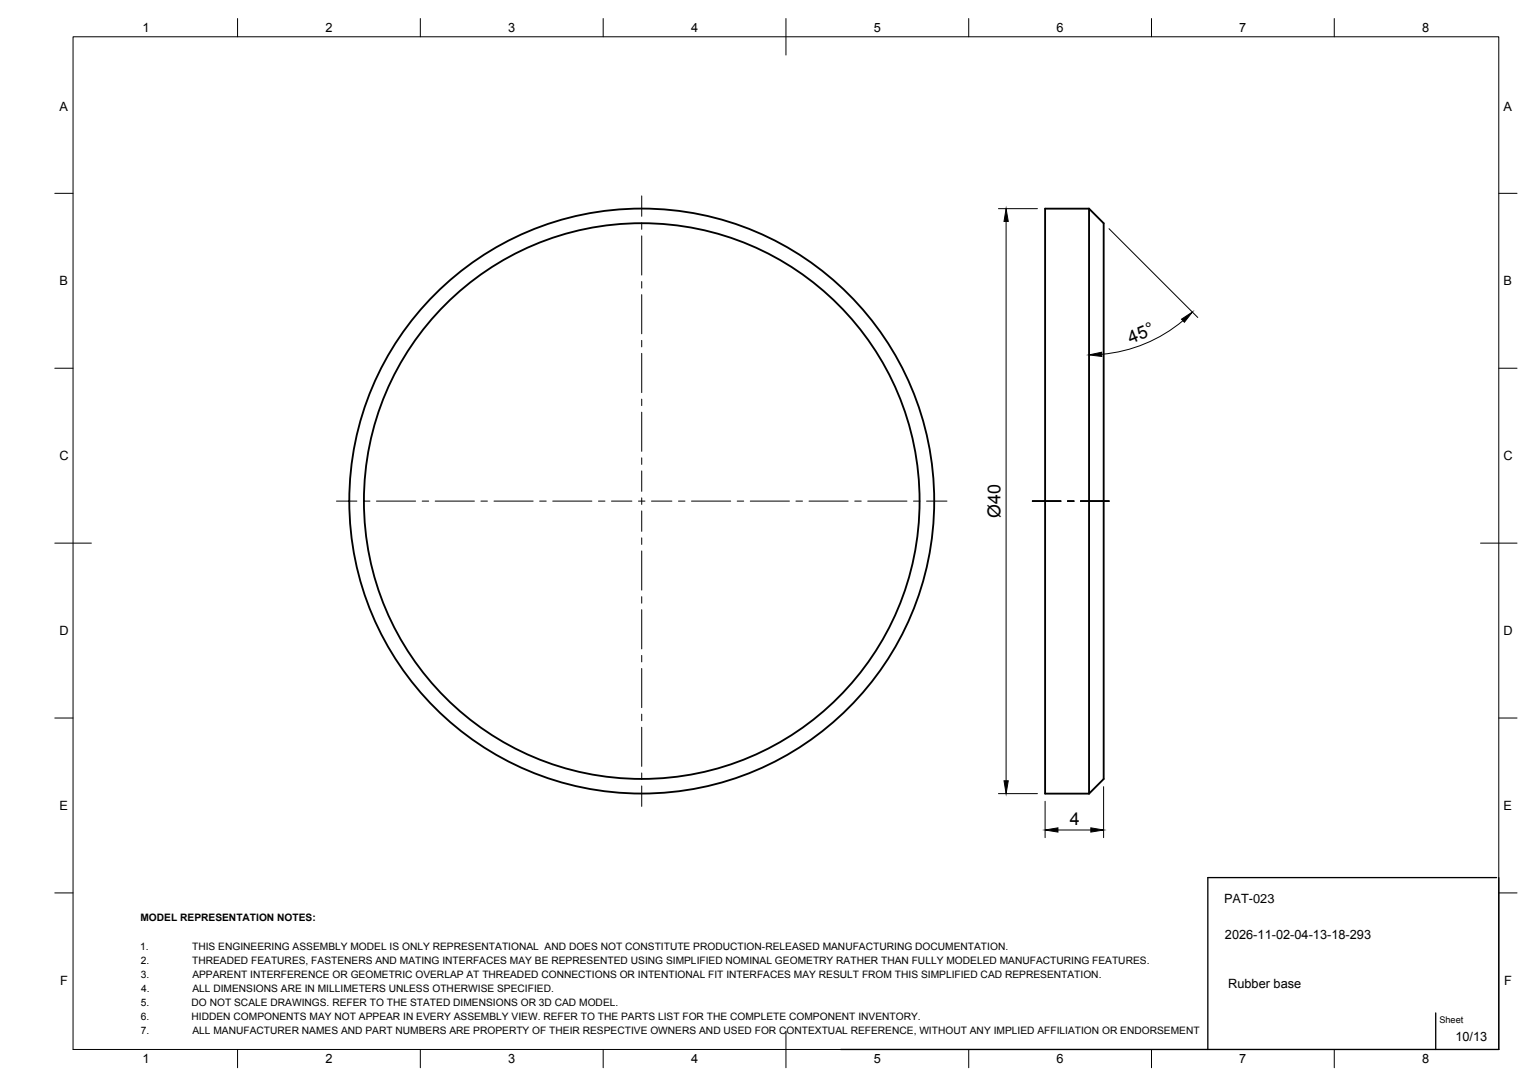
ISO-10303-21;
HEADER;
/* Generated by software containing ST-Developer
 * from STEP Tools, Inc. (www.steptools.com) 
 */

FILE_DESCRIPTION(
/* description */ ('PAT-023'),
/* implementation_level */ '2;1');

FILE_NAME(
/* name */ 'Rubber base.step',
/* time_stamp */ '2026-10-29T15:47:46-07:00',
/* author */ (''),
/* organization */ (''),
/* preprocessor_version */ 'ST-DEVELOPER v20.2',
/* originating_system */ 'Autodesk Translation Framework v15.17.0.0',
/* authorisation */ '');

FILE_SCHEMA (('AUTOMOTIVE_DESIGN { 1 0 10303 214 3 1 1 }'));
ENDSEC;

DATA;
#10=MECHANICAL_DESIGN_GEOMETRIC_PRESENTATION_REPRESENTATION('',(#87),#3773);
#63=CONICAL_SURFACE('',#2387,1.95,0.785398163397449);
#71=SHAPE_REPRESENTATION_RELATIONSHIP('SRR','None',#3819,#79);
#79=ADVANCED_BREP_SHAPE_REPRESENTATION('',(#95),#3767);
#87=STYLED_ITEM('',(#3953),#95);
#95=MANIFOLD_SOLID_BREP('Body1',#2240);
#150=PLANE('',#2385);
#151=PLANE('',#2391);
#256=FACE_OUTER_BOUND('',#384,.T.);
#257=FACE_OUTER_BOUND('',#385,.T.);
#258=FACE_OUTER_BOUND('',#386,.T.);
#259=FACE_OUTER_BOUND('',#387,.T.);
#384=EDGE_LOOP('',(#1711));
#385=EDGE_LOOP('',(#1712,#1713,#1714,#1715));
#386=EDGE_LOOP('',(#1716,#1717,#1718,#1719));
#387=EDGE_LOOP('',(#1720));
#562=LINE('',#3314,#826);
#563=LINE('',#3318,#827);
#826=VECTOR('',#2703,1.95);
#827=VECTOR('',#2708,2.);
#1005=CIRCLE('',#2386,1.9);
#1006=CIRCLE('',#2388,2.);
#1007=CIRCLE('',#2390,2.);
#1089=VERTEX_POINT('',#3309);
#1090=VERTEX_POINT('',#3312);
#1091=VERTEX_POINT('',#3316);
#1318=EDGE_CURVE('',#1089,#1089,#1005,.T.);
#1319=EDGE_CURVE('',#1090,#1090,#1006,.T.);
#1320=EDGE_CURVE('',#1090,#1089,#562,.T.);
#1321=EDGE_CURVE('',#1091,#1091,#1007,.T.);
#1322=EDGE_CURVE('',#1091,#1090,#563,.T.);
#1711=ORIENTED_EDGE('',*,*,#1318,.F.);
#1712=ORIENTED_EDGE('',*,*,#1319,.F.);
#1713=ORIENTED_EDGE('',*,*,#1320,.T.);
#1714=ORIENTED_EDGE('',*,*,#1318,.T.);
#1715=ORIENTED_EDGE('',*,*,#1320,.F.);
#1716=ORIENTED_EDGE('',*,*,#1321,.F.);
#1717=ORIENTED_EDGE('',*,*,#1322,.T.);
#1718=ORIENTED_EDGE('',*,*,#1319,.T.);
#1719=ORIENTED_EDGE('',*,*,#1322,.F.);
#1720=ORIENTED_EDGE('',*,*,#1321,.T.);
#2112=CYLINDRICAL_SURFACE('',#2389,2.);
#2156=ADVANCED_FACE('',(#256),#150,.T.);
#2157=ADVANCED_FACE('',(#257),#63,.T.);
#2158=ADVANCED_FACE('',(#258),#2112,.T.);
#2159=ADVANCED_FACE('',(#259),#151,.T.);
#2240=CLOSED_SHELL('',(#2156,#2157,#2158,#2159));
#2384=AXIS2_PLACEMENT_3D('',#3307,#2693,#2694);
#2385=AXIS2_PLACEMENT_3D('',#3308,#2695,#2696);
#2386=AXIS2_PLACEMENT_3D('',#3310,#2697,#2698);
#2387=AXIS2_PLACEMENT_3D('',#3311,#2699,#2700);
#2388=AXIS2_PLACEMENT_3D('',#3313,#2701,#2702);
#2389=AXIS2_PLACEMENT_3D('',#3315,#2704,#2705);
#2390=AXIS2_PLACEMENT_3D('',#3317,#2706,#2707);
#2391=AXIS2_PLACEMENT_3D('',#3319,#2709,#2710);
#2693=DIRECTION('axis',(0.,0.,1.));
#2694=DIRECTION('refdir',(1.,0.,0.));
#2695=DIRECTION('center_axis',(0.,0.,-1.));
#2696=DIRECTION('ref_axis',(-1.,0.,0.));
#2697=DIRECTION('center_axis',(0.,0.,1.));
#2698=DIRECTION('ref_axis',(1.,0.,0.));
#2699=DIRECTION('center_axis',(0.,0.,1.));
#2700=DIRECTION('ref_axis',(1.,0.,0.));
#2701=DIRECTION('center_axis',(0.,0.,1.));
#2702=DIRECTION('ref_axis',(1.,0.,0.));
#2703=DIRECTION('',(0.707106781186548,8.65956056235494E-17,-0.707106781186547));
#2704=DIRECTION('center_axis',(0.,0.,1.));
#2705=DIRECTION('ref_axis',(1.,0.,0.));
#2706=DIRECTION('center_axis',(0.,0.,1.));
#2707=DIRECTION('ref_axis',(1.,0.,0.));
#2708=DIRECTION('',(0.,0.,-1.));
#2709=DIRECTION('center_axis',(0.,0.,1.));
#2710=DIRECTION('ref_axis',(1.,0.,0.));
#3307=CARTESIAN_POINT('',(0.,0.,0.));
#3308=CARTESIAN_POINT('Origin',(1.9,0.,0.));
#3309=CARTESIAN_POINT('',(-1.9,-2.32682891837997E-16,-4.16333634234434E-17));
#3310=CARTESIAN_POINT('Origin',(0.,0.,0.));
#3311=CARTESIAN_POINT('Origin',(0.,0.,0.05));
#3312=CARTESIAN_POINT('',(-2.,-2.44929359829471E-16,0.1));
#3313=CARTESIAN_POINT('Origin',(0.,0.,0.1));
#3314=CARTESIAN_POINT('',(-1.95,-2.38806125833734E-16,0.05));
#3315=CARTESIAN_POINT('Origin',(0.,0.,0.25));
#3316=CARTESIAN_POINT('',(-2.,-2.44929359829471E-16,0.4));
#3317=CARTESIAN_POINT('Origin',(0.,0.,0.4));
#3318=CARTESIAN_POINT('',(-2.,-2.44929359829471E-16,0.25));
#3319=CARTESIAN_POINT('Origin',(0.,0.,0.4));
#3754=UNCERTAINTY_MEASURE_WITH_UNIT(LENGTH_MEASURE(0.001),#3774,
'DISTANCE_ACCURACY_VALUE',
'Maximum model space distance between geometric entities at asserted c
onnectivities');
#3760=UNCERTAINTY_MEASURE_WITH_UNIT(LENGTH_MEASURE(0.001),#3774,
'DISTANCE_ACCURACY_VALUE',
'Maximum model space distance between geometric entities at asserted c
onnectivities');
#3767=(
GEOMETRIC_REPRESENTATION_CONTEXT(3)
GLOBAL_UNCERTAINTY_ASSIGNED_CONTEXT((#3754))
GLOBAL_UNIT_ASSIGNED_CONTEXT((#3774,#3776,#3777))
REPRESENTATION_CONTEXT('','3D')
);
#3773=(
GEOMETRIC_REPRESENTATION_CONTEXT(3)
GLOBAL_UNCERTAINTY_ASSIGNED_CONTEXT((#3760))
GLOBAL_UNIT_ASSIGNED_CONTEXT((#3774,#3776,#3777))
REPRESENTATION_CONTEXT('','3D')
);
#3774=(
LENGTH_UNIT()
NAMED_UNIT(*)
SI_UNIT(.CENTI.,.METRE.)
);
#3776=(
NAMED_UNIT(*)
PLANE_ANGLE_UNIT()
SI_UNIT($,.RADIAN.)
);
#3777=(
NAMED_UNIT(*)
SI_UNIT($,.STERADIAN.)
SOLID_ANGLE_UNIT()
);
#3784=SHAPE_DEFINITION_REPRESENTATION(#3796,#3819);
#3796=PRODUCT_DEFINITION_SHAPE('',$,#3832);
#3819=SHAPE_REPRESENTATION('',(#2384),#3767);
#3825=PRODUCT_DEFINITION_CONTEXT('part definition',#3863,'design');
#3832=PRODUCT_DEFINITION('Rubber base','Rubber base',#3844,
#3825);
#3844=PRODUCT_DEFINITION_FORMATION('',$,#3871);
#3863=APPLICATION_CONTEXT(
'Core Data for Automotive Mechanical Design Process');
#3864=PRODUCT_CONTEXT('part definition',#3863,'mechanical');
#3871=PRODUCT('Rubber base','Rubber base','Rubber base',(#3864));
#3947=COLOUR_RGB('Black',0.12,0.14,0.17);
#3948=FILL_AREA_STYLE_COLOUR('',#3947);
#3949=FILL_AREA_STYLE('',(#3948));
#3950=SURFACE_STYLE_FILL_AREA(#3949);
#3951=SURFACE_SIDE_STYLE('',(#3950));
#3952=SURFACE_STYLE_USAGE(.BOTH.,#3951);
#3953=PRESENTATION_STYLE_ASSIGNMENT((#3952));
ENDSEC;
END-ISO-10303-21;
